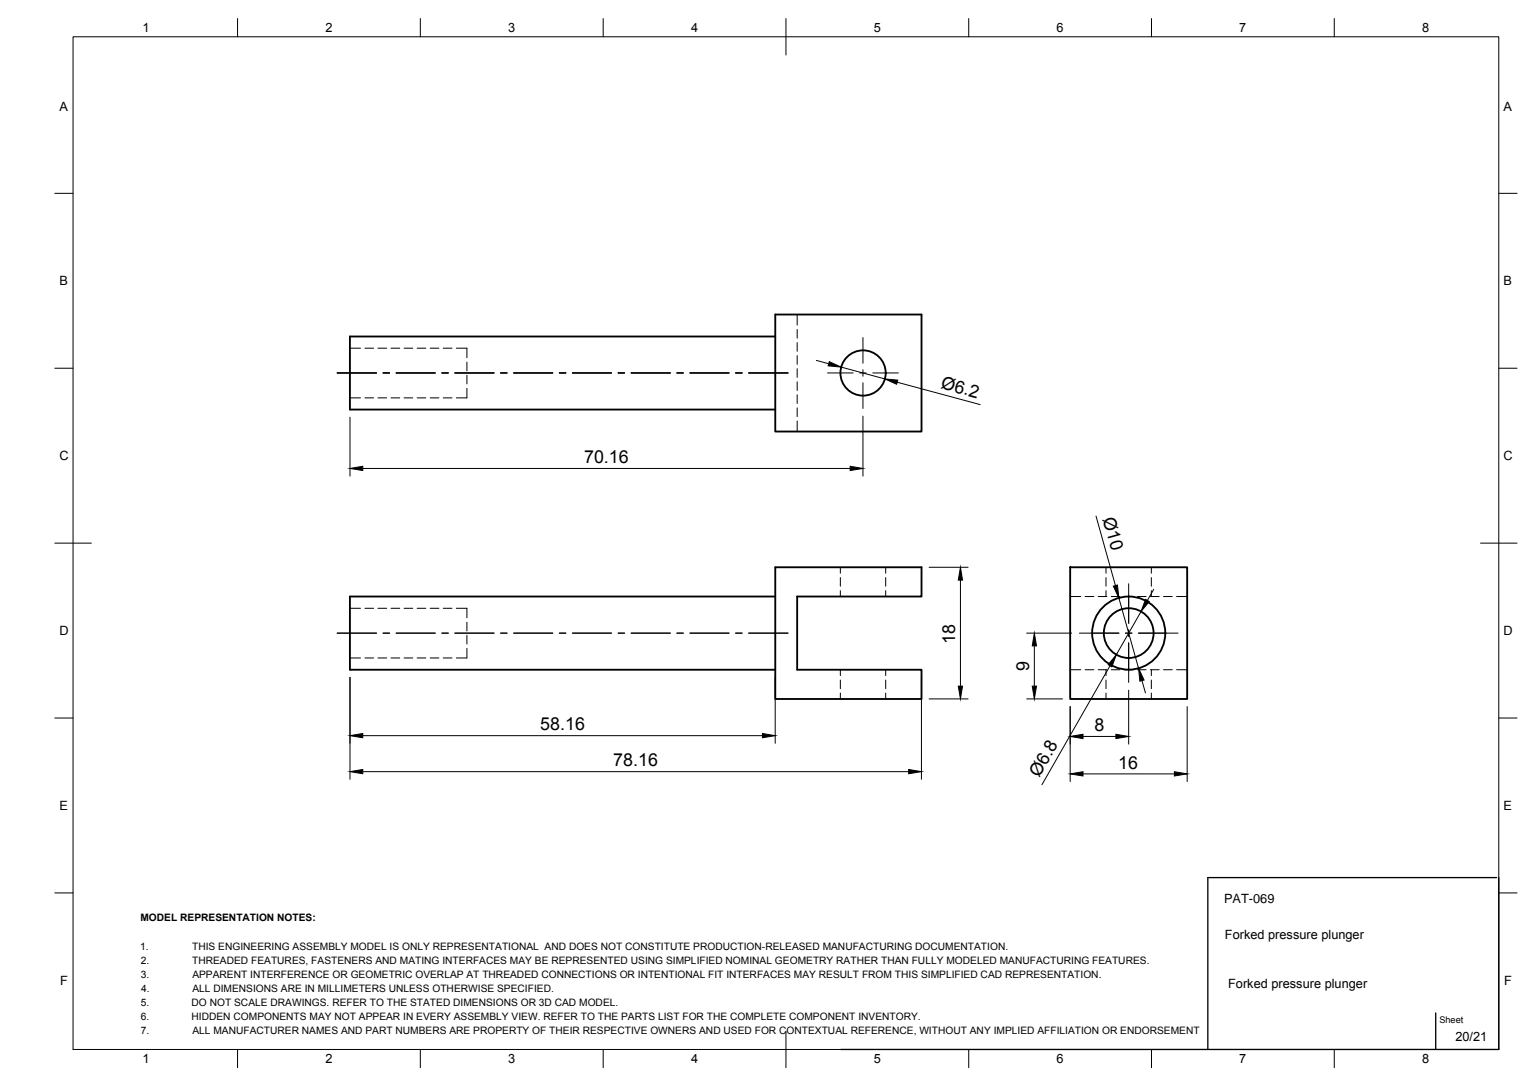
ISO-10303-21;
HEADER;
/* Generated by software containing ST-Developer
 * from STEP Tools, Inc. (www.steptools.com) 
 */

FILE_DESCRIPTION(
/* description */ ('Located fixture plate with toggle clamp'),
/* implementation_level */ '2;1');

FILE_NAME(
/* name */ 'Forked pressure plunger.step',
/* time_stamp */ '2026-10-27T21:36:12-07:00',
/* author */ (''),
/* organization */ (''),
/* preprocessor_version */ 'ST-DEVELOPER v20.2',
/* originating_system */ 'Autodesk Translation Framework v15.17.0.0',
/* authorisation */ '');

FILE_SCHEMA (('AUTOMOTIVE_DESIGN { 1 0 10303 214 3 1 1 }'));
ENDSEC;

DATA;
#10=MECHANICAL_DESIGN_GEOMETRIC_PRESENTATION_REPRESENTATION('',(#337),#9285);
#289=SHAPE_REPRESENTATION_RELATIONSHIP('SRR','None',#9415,#313);
#313=ADVANCED_BREP_SHAPE_REPRESENTATION('',(#358),#9277);
#337=STYLED_ITEM('',(#9598),#358);
#358=MANIFOLD_SOLID_BREP('Body1',#5188);
#470=FACE_BOUND('',#1310,.T.);
#471=FACE_BOUND('',#1313,.T.);
#472=FACE_BOUND('',#1316,.T.);
#473=FACE_BOUND('',#1319,.T.);
#474=FACE_BOUND('',#1322,.T.);
#475=FACE_BOUND('',#1325,.T.);
#632=PLANE('',#5880);
#633=PLANE('',#5887);
#634=PLANE('',#5888);
#635=PLANE('',#5889);
#636=PLANE('',#5890);
#637=PLANE('',#5891);
#638=PLANE('',#5892);
#639=PLANE('',#5894);
#640=PLANE('',#5895);
#641=PLANE('',#5896);
#642=PLANE('',#5897);
#643=PLANE('',#5900);
#905=FACE_OUTER_BOUND('',#1304,.T.);
#906=FACE_OUTER_BOUND('',#1305,.T.);
#907=FACE_OUTER_BOUND('',#1306,.T.);
#908=FACE_OUTER_BOUND('',#1307,.T.);
#909=FACE_OUTER_BOUND('',#1308,.T.);
#910=FACE_OUTER_BOUND('',#1309,.T.);
#911=FACE_OUTER_BOUND('',#1311,.T.);
#912=FACE_OUTER_BOUND('',#1312,.T.);
#913=FACE_OUTER_BOUND('',#1314,.T.);
#914=FACE_OUTER_BOUND('',#1315,.T.);
#915=FACE_OUTER_BOUND('',#1317,.T.);
#916=FACE_OUTER_BOUND('',#1318,.T.);
#917=FACE_OUTER_BOUND('',#1320,.T.);
#918=FACE_OUTER_BOUND('',#1321,.T.);
#919=FACE_OUTER_BOUND('',#1323,.T.);
#920=FACE_OUTER_BOUND('',#1324,.T.);
#1304=EDGE_LOOP('',(#4534,#4535,#4536,#4537));
#1305=EDGE_LOOP('',(#4538));
#1306=EDGE_LOOP('',(#4539,#4540,#4541,#4542));
#1307=EDGE_LOOP('',(#4543,#4544,#4545,#4546));
#1308=EDGE_LOOP('',(#4547,#4548,#4549,#4550));
#1309=EDGE_LOOP('',(#4551,#4552,#4553,#4554));
#1310=EDGE_LOOP('',(#4555));
#1311=EDGE_LOOP('',(#4556,#4557,#4558,#4559,#4560,#4561,#4562,#4563));
#1312=EDGE_LOOP('',(#4564,#4565,#4566,#4567));
#1313=EDGE_LOOP('',(#4568));
#1314=EDGE_LOOP('',(#4569,#4570,#4571,#4572));
#1315=EDGE_LOOP('',(#4573,#4574,#4575,#4576));
#1316=EDGE_LOOP('',(#4577));
#1317=EDGE_LOOP('',(#4578,#4579,#4580,#4581,#4582,#4583,#4584,#4585));
#1318=EDGE_LOOP('',(#4586,#4587,#4588,#4589));
#1319=EDGE_LOOP('',(#4590));
#1320=EDGE_LOOP('',(#4591,#4592,#4593,#4594));
#1321=EDGE_LOOP('',(#4595,#4596,#4597,#4598));
#1322=EDGE_LOOP('',(#4599));
#1323=EDGE_LOOP('',(#4600,#4601,#4602,#4603));
#1324=EDGE_LOOP('',(#4604));
#1325=EDGE_LOOP('',(#4605));
#1544=CIRCLE('',#5878,0.34);
#1545=CIRCLE('',#5879,0.34);
#1546=CIRCLE('',#5882,0.31);
#1547=CIRCLE('',#5883,0.31);
#1548=CIRCLE('',#5885,0.31);
#1549=CIRCLE('',#5886,0.31);
#1550=CIRCLE('',#5893,0.5);
#1551=CIRCLE('',#5899,0.5);
#1923=LINE('',#8748,#2333);
#1924=LINE('',#8755,#2334);
#1925=LINE('',#8761,#2335);
#1926=LINE('',#8766,#2336);
#1927=LINE('',#8768,#2337);
#1928=LINE('',#8770,#2338);
#1929=LINE('',#8771,#2339);
#1930=LINE('',#8775,#2340);
#1931=LINE('',#8777,#2341);
#1932=LINE('',#8779,#2342);
#1933=LINE('',#8780,#2343);
#1934=LINE('',#8783,#2344);
#1935=LINE('',#8784,#2345);
#1936=LINE('',#8786,#2346);
#1937=LINE('',#8788,#2347);
#1938=LINE('',#8790,#2348);
#1939=LINE('',#8791,#2349);
#1940=LINE('',#8795,#2350);
#1941=LINE('',#8796,#2351);
#1942=LINE('',#8797,#2352);
#1943=LINE('',#8800,#2353);
#1944=LINE('',#8801,#2354);
#1945=LINE('',#8803,#2355);
#1946=LINE('',#8807,#2356);
#1947=LINE('',#8809,#2357);
#1948=LINE('',#8810,#2358);
#1949=LINE('',#8813,#2359);
#1950=LINE('',#8818,#2360);
#2333=VECTOR('',#7207,0.34);
#2334=VECTOR('',#7216,0.31);
#2335=VECTOR('',#7223,0.31);
#2336=VECTOR('',#7228,1.);
#2337=VECTOR('',#7229,1.);
#2338=VECTOR('',#7230,1.);
#2339=VECTOR('',#7231,1.);
#2340=VECTOR('',#7234,1.);
#2341=VECTOR('',#7235,1.);
#2342=VECTOR('',#7236,1.);
#2343=VECTOR('',#7237,1.);
#2344=VECTOR('',#7240,1.);
#2345=VECTOR('',#7241,1.);
#2346=VECTOR('',#7242,1.);
#2347=VECTOR('',#7243,1.);
#2348=VECTOR('',#7244,1.);
#2349=VECTOR('',#7245,1.);
#2350=VECTOR('',#7248,1.);
#2351=VECTOR('',#7249,1.);
#2352=VECTOR('',#7250,1.);
#2353=VECTOR('',#7253,1.);
#2354=VECTOR('',#7254,1.);
#2355=VECTOR('',#7257,1.);
#2356=VECTOR('',#7262,1.);
#2357=VECTOR('',#7263,1.);
#2358=VECTOR('',#7264,1.);
#2359=VECTOR('',#7269,1.);
#2360=VECTOR('',#7276,0.5);
#2746=VERTEX_POINT('',#8745);
#2747=VERTEX_POINT('',#8747);
#2748=VERTEX_POINT('',#8752);
#2749=VERTEX_POINT('',#8754);
#2750=VERTEX_POINT('',#8758);
#2751=VERTEX_POINT('',#8760);
#2752=VERTEX_POINT('',#8764);
#2753=VERTEX_POINT('',#8765);
#2754=VERTEX_POINT('',#8767);
#2755=VERTEX_POINT('',#8769);
#2756=VERTEX_POINT('',#8773);
#2757=VERTEX_POINT('',#8774);
#2758=VERTEX_POINT('',#8776);
#2759=VERTEX_POINT('',#8778);
#2760=VERTEX_POINT('',#8782);
#2761=VERTEX_POINT('',#8785);
#2762=VERTEX_POINT('',#8787);
#2763=VERTEX_POINT('',#8789);
#2764=VERTEX_POINT('',#8793);
#2765=VERTEX_POINT('',#8794);
#2766=VERTEX_POINT('',#8799);
#2767=VERTEX_POINT('',#8804);
#2768=VERTEX_POINT('',#8808);
#2769=VERTEX_POINT('',#8816);
#3355=EDGE_CURVE('',#2746,#2746,#1544,.T.);
#3356=EDGE_CURVE('',#2746,#2747,#1923,.T.);
#3357=EDGE_CURVE('',#2747,#2747,#1545,.T.);
#3358=EDGE_CURVE('',#2748,#2748,#1546,.T.);
#3359=EDGE_CURVE('',#2748,#2749,#1924,.T.);
#3360=EDGE_CURVE('',#2749,#2749,#1547,.T.);
#3361=EDGE_CURVE('',#2750,#2750,#1548,.T.);
#3362=EDGE_CURVE('',#2750,#2751,#1925,.T.);
#3363=EDGE_CURVE('',#2751,#2751,#1549,.T.);
#3364=EDGE_CURVE('',#2752,#2753,#1926,.T.);
#3365=EDGE_CURVE('',#2754,#2752,#1927,.T.);
#3366=EDGE_CURVE('',#2755,#2754,#1928,.T.);
#3367=EDGE_CURVE('',#2755,#2753,#1929,.T.);
#3368=EDGE_CURVE('',#2756,#2757,#1930,.T.);
#3369=EDGE_CURVE('',#2757,#2758,#1931,.T.);
#3370=EDGE_CURVE('',#2758,#2759,#1932,.T.);
#3371=EDGE_CURVE('',#2759,#2756,#1933,.T.);
#3372=EDGE_CURVE('',#2760,#2752,#1934,.T.);
#3373=EDGE_CURVE('',#2760,#2757,#1935,.T.);
#3374=EDGE_CURVE('',#2761,#2756,#1936,.T.);
#3375=EDGE_CURVE('',#2762,#2761,#1937,.T.);
#3376=EDGE_CURVE('',#2762,#2763,#1938,.T.);
#3377=EDGE_CURVE('',#2754,#2763,#1939,.T.);
#3378=EDGE_CURVE('',#2764,#2765,#1940,.T.);
#3379=EDGE_CURVE('',#2765,#2762,#1941,.T.);
#3380=EDGE_CURVE('',#2761,#2764,#1942,.T.);
#3381=EDGE_CURVE('',#2766,#2760,#1943,.T.);
#3382=EDGE_CURVE('',#2766,#2758,#1944,.T.);
#3383=EDGE_CURVE('',#2764,#2759,#1945,.T.);
#3384=EDGE_CURVE('',#2767,#2767,#1550,.T.);
#3385=EDGE_CURVE('',#2753,#2766,#1946,.T.);
#3386=EDGE_CURVE('',#2768,#2755,#1947,.T.);
#3387=EDGE_CURVE('',#2765,#2768,#1948,.T.);
#3388=EDGE_CURVE('',#2763,#2768,#1949,.T.);
#3389=EDGE_CURVE('',#2769,#2769,#1551,.T.);
#3390=EDGE_CURVE('',#2769,#2767,#1950,.T.);
#4534=ORIENTED_EDGE('',*,*,#3355,.F.);
#4535=ORIENTED_EDGE('',*,*,#3356,.T.);
#4536=ORIENTED_EDGE('',*,*,#3357,.F.);
#4537=ORIENTED_EDGE('',*,*,#3356,.F.);
#4538=ORIENTED_EDGE('',*,*,#3355,.T.);
#4539=ORIENTED_EDGE('',*,*,#3358,.F.);
#4540=ORIENTED_EDGE('',*,*,#3359,.T.);
#4541=ORIENTED_EDGE('',*,*,#3360,.F.);
#4542=ORIENTED_EDGE('',*,*,#3359,.F.);
#4543=ORIENTED_EDGE('',*,*,#3361,.F.);
#4544=ORIENTED_EDGE('',*,*,#3362,.T.);
#4545=ORIENTED_EDGE('',*,*,#3363,.F.);
#4546=ORIENTED_EDGE('',*,*,#3362,.F.);
#4547=ORIENTED_EDGE('',*,*,#3364,.F.);
#4548=ORIENTED_EDGE('',*,*,#3365,.F.);
#4549=ORIENTED_EDGE('',*,*,#3366,.F.);
#4550=ORIENTED_EDGE('',*,*,#3367,.T.);
#4551=ORIENTED_EDGE('',*,*,#3368,.T.);
#4552=ORIENTED_EDGE('',*,*,#3369,.T.);
#4553=ORIENTED_EDGE('',*,*,#3370,.T.);
#4554=ORIENTED_EDGE('',*,*,#3371,.T.);
#4555=ORIENTED_EDGE('',*,*,#3363,.T.);
#4556=ORIENTED_EDGE('',*,*,#3372,.F.);
#4557=ORIENTED_EDGE('',*,*,#3373,.T.);
#4558=ORIENTED_EDGE('',*,*,#3368,.F.);
#4559=ORIENTED_EDGE('',*,*,#3374,.F.);
#4560=ORIENTED_EDGE('',*,*,#3375,.F.);
#4561=ORIENTED_EDGE('',*,*,#3376,.T.);
#4562=ORIENTED_EDGE('',*,*,#3377,.F.);
#4563=ORIENTED_EDGE('',*,*,#3365,.T.);
#4564=ORIENTED_EDGE('',*,*,#3378,.T.);
#4565=ORIENTED_EDGE('',*,*,#3379,.T.);
#4566=ORIENTED_EDGE('',*,*,#3375,.T.);
#4567=ORIENTED_EDGE('',*,*,#3380,.T.);
#4568=ORIENTED_EDGE('',*,*,#3358,.T.);
#4569=ORIENTED_EDGE('',*,*,#3381,.F.);
#4570=ORIENTED_EDGE('',*,*,#3382,.T.);
#4571=ORIENTED_EDGE('',*,*,#3369,.F.);
#4572=ORIENTED_EDGE('',*,*,#3373,.F.);
#4573=ORIENTED_EDGE('',*,*,#3374,.T.);
#4574=ORIENTED_EDGE('',*,*,#3371,.F.);
#4575=ORIENTED_EDGE('',*,*,#3383,.F.);
#4576=ORIENTED_EDGE('',*,*,#3380,.F.);
#4577=ORIENTED_EDGE('',*,*,#3384,.F.);
#4578=ORIENTED_EDGE('',*,*,#3370,.F.);
#4579=ORIENTED_EDGE('',*,*,#3382,.F.);
#4580=ORIENTED_EDGE('',*,*,#3385,.F.);
#4581=ORIENTED_EDGE('',*,*,#3367,.F.);
#4582=ORIENTED_EDGE('',*,*,#3386,.F.);
#4583=ORIENTED_EDGE('',*,*,#3387,.F.);
#4584=ORIENTED_EDGE('',*,*,#3378,.F.);
#4585=ORIENTED_EDGE('',*,*,#3383,.T.);
#4586=ORIENTED_EDGE('',*,*,#3364,.T.);
#4587=ORIENTED_EDGE('',*,*,#3385,.T.);
#4588=ORIENTED_EDGE('',*,*,#3381,.T.);
#4589=ORIENTED_EDGE('',*,*,#3372,.T.);
#4590=ORIENTED_EDGE('',*,*,#3361,.T.);
#4591=ORIENTED_EDGE('',*,*,#3379,.F.);
#4592=ORIENTED_EDGE('',*,*,#3387,.T.);
#4593=ORIENTED_EDGE('',*,*,#3388,.F.);
#4594=ORIENTED_EDGE('',*,*,#3376,.F.);
#4595=ORIENTED_EDGE('',*,*,#3366,.T.);
#4596=ORIENTED_EDGE('',*,*,#3377,.T.);
#4597=ORIENTED_EDGE('',*,*,#3388,.T.);
#4598=ORIENTED_EDGE('',*,*,#3386,.T.);
#4599=ORIENTED_EDGE('',*,*,#3360,.T.);
#4600=ORIENTED_EDGE('',*,*,#3389,.F.);
#4601=ORIENTED_EDGE('',*,*,#3390,.T.);
#4602=ORIENTED_EDGE('',*,*,#3384,.T.);
#4603=ORIENTED_EDGE('',*,*,#3390,.F.);
#4604=ORIENTED_EDGE('',*,*,#3389,.T.);
#4605=ORIENTED_EDGE('',*,*,#3357,.T.);
#4859=CYLINDRICAL_SURFACE('',#5877,0.34);
#4860=CYLINDRICAL_SURFACE('',#5881,0.31);
#4861=CYLINDRICAL_SURFACE('',#5884,0.31);
#4862=CYLINDRICAL_SURFACE('',#5898,0.5);
#5106=ADVANCED_FACE('',(#905),#4859,.F.);
#5107=ADVANCED_FACE('',(#906),#632,.T.);
#5108=ADVANCED_FACE('',(#907),#4860,.F.);
#5109=ADVANCED_FACE('',(#908),#4861,.F.);
#5110=ADVANCED_FACE('',(#909),#633,.T.);
#5111=ADVANCED_FACE('',(#910,#470),#634,.T.);
#5112=ADVANCED_FACE('',(#911),#635,.T.);
#5113=ADVANCED_FACE('',(#912,#471),#636,.F.);
#5114=ADVANCED_FACE('',(#913),#637,.T.);
#5115=ADVANCED_FACE('',(#914,#472),#638,.T.);
#5116=ADVANCED_FACE('',(#915),#639,.T.);
#5117=ADVANCED_FACE('',(#916,#473),#640,.F.);
#5118=ADVANCED_FACE('',(#917),#641,.T.);
#5119=ADVANCED_FACE('',(#918,#474),#642,.T.);
#5120=ADVANCED_FACE('',(#919),#4862,.T.);
#5121=ADVANCED_FACE('',(#920,#475),#643,.T.);
#5188=CLOSED_SHELL('',(#5106,#5107,#5108,#5109,#5110,#5111,#5112,#5113,
#5114,#5115,#5116,#5117,#5118,#5119,#5120,#5121));
#5876=AXIS2_PLACEMENT_3D('',#8743,#7201,#7202);
#5877=AXIS2_PLACEMENT_3D('',#8744,#7203,#7204);
#5878=AXIS2_PLACEMENT_3D('',#8746,#7205,#7206);
#5879=AXIS2_PLACEMENT_3D('',#8749,#7208,#7209);
#5880=AXIS2_PLACEMENT_3D('',#8750,#7210,#7211);
#5881=AXIS2_PLACEMENT_3D('',#8751,#7212,#7213);
#5882=AXIS2_PLACEMENT_3D('',#8753,#7214,#7215);
#5883=AXIS2_PLACEMENT_3D('',#8756,#7217,#7218);
#5884=AXIS2_PLACEMENT_3D('',#8757,#7219,#7220);
#5885=AXIS2_PLACEMENT_3D('',#8759,#7221,#7222);
#5886=AXIS2_PLACEMENT_3D('',#8762,#7224,#7225);
#5887=AXIS2_PLACEMENT_3D('',#8763,#7226,#7227);
#5888=AXIS2_PLACEMENT_3D('',#8772,#7232,#7233);
#5889=AXIS2_PLACEMENT_3D('',#8781,#7238,#7239);
#5890=AXIS2_PLACEMENT_3D('',#8792,#7246,#7247);
#5891=AXIS2_PLACEMENT_3D('',#8798,#7251,#7252);
#5892=AXIS2_PLACEMENT_3D('',#8802,#7255,#7256);
#5893=AXIS2_PLACEMENT_3D('',#8805,#7258,#7259);
#5894=AXIS2_PLACEMENT_3D('',#8806,#7260,#7261);
#5895=AXIS2_PLACEMENT_3D('',#8811,#7265,#7266);
#5896=AXIS2_PLACEMENT_3D('',#8812,#7267,#7268);
#5897=AXIS2_PLACEMENT_3D('',#8814,#7270,#7271);
#5898=AXIS2_PLACEMENT_3D('',#8815,#7272,#7273);
#5899=AXIS2_PLACEMENT_3D('',#8817,#7274,#7275);
#5900=AXIS2_PLACEMENT_3D('',#8819,#7277,#7278);
#7201=DIRECTION('axis',(0.,0.,1.));
#7202=DIRECTION('refdir',(1.,0.,0.));
#7203=DIRECTION('center_axis',(1.,0.,0.));
#7204=DIRECTION('ref_axis',(0.,0.,-1.));
#7205=DIRECTION('center_axis',(1.,0.,0.));
#7206=DIRECTION('ref_axis',(0.,0.,-1.));
#7207=DIRECTION('',(1.,0.,0.));
#7208=DIRECTION('center_axis',(-1.,0.,0.));
#7209=DIRECTION('ref_axis',(0.,0.,-1.));
#7210=DIRECTION('center_axis',(1.,0.,0.));
#7211=DIRECTION('ref_axis',(0.,0.,-1.));
#7212=DIRECTION('center_axis',(0.,1.,0.));
#7213=DIRECTION('ref_axis',(1.,0.,0.));
#7214=DIRECTION('center_axis',(0.,1.,0.));
#7215=DIRECTION('ref_axis',(1.,0.,0.));
#7216=DIRECTION('',(0.,1.,0.));
#7217=DIRECTION('center_axis',(0.,-1.,0.));
#7218=DIRECTION('ref_axis',(1.,0.,0.));
#7219=DIRECTION('center_axis',(0.,1.,0.));
#7220=DIRECTION('ref_axis',(1.,0.,0.));
#7221=DIRECTION('center_axis',(0.,1.,0.));
#7222=DIRECTION('ref_axis',(1.,0.,0.));
#7223=DIRECTION('',(0.,1.,0.));
#7224=DIRECTION('center_axis',(0.,-1.,0.));
#7225=DIRECTION('ref_axis',(1.,0.,0.));
#7226=DIRECTION('center_axis',(-1.,0.,0.));
#7227=DIRECTION('ref_axis',(0.,0.,1.));
#7228=DIRECTION('',(0.,0.,1.));
#7229=DIRECTION('',(0.,1.,0.));
#7230=DIRECTION('',(0.,0.,-1.));
#7231=DIRECTION('',(0.,1.,0.));
#7232=DIRECTION('center_axis',(0.,1.,0.));
#7233=DIRECTION('ref_axis',(0.,0.,1.));
#7234=DIRECTION('',(-1.,0.,0.));
#7235=DIRECTION('',(0.,0.,1.));
#7236=DIRECTION('',(1.,0.,0.));
#7237=DIRECTION('',(0.,0.,-1.));
#7238=DIRECTION('center_axis',(0.,0.,-1.));
#7239=DIRECTION('ref_axis',(-1.,0.,0.));
#7240=DIRECTION('',(1.,0.,0.));
#7241=DIRECTION('',(0.,1.,0.));
#7242=DIRECTION('',(0.,1.,0.));
#7243=DIRECTION('',(1.,0.,0.));
#7244=DIRECTION('',(0.,1.,0.));
#7245=DIRECTION('',(-1.,0.,0.));
#7246=DIRECTION('center_axis',(0.,1.,0.));
#7247=DIRECTION('ref_axis',(1.,0.,0.));
#7248=DIRECTION('',(-1.,0.,0.));
#7249=DIRECTION('',(0.,0.,-1.));
#7250=DIRECTION('',(0.,0.,1.));
#7251=DIRECTION('center_axis',(-1.,0.,0.));
#7252=DIRECTION('ref_axis',(0.,0.,1.));
#7253=DIRECTION('',(0.,0.,-1.));
#7254=DIRECTION('',(0.,1.,0.));
#7255=DIRECTION('center_axis',(1.,0.,0.));
#7256=DIRECTION('ref_axis',(0.,0.,-1.));
#7257=DIRECTION('',(0.,1.,0.));
#7258=DIRECTION('center_axis',(1.,0.,0.));
#7259=DIRECTION('ref_axis',(0.,0.,-1.));
#7260=DIRECTION('center_axis',(0.,0.,1.));
#7261=DIRECTION('ref_axis',(1.,0.,0.));
#7262=DIRECTION('',(-1.,0.,0.));
#7263=DIRECTION('',(1.,0.,0.));
#7264=DIRECTION('',(0.,1.,0.));
#7265=DIRECTION('center_axis',(0.,1.,0.));
#7266=DIRECTION('ref_axis',(1.,0.,0.));
#7267=DIRECTION('center_axis',(-1.,0.,0.));
#7268=DIRECTION('ref_axis',(0.,0.,1.));
#7269=DIRECTION('',(0.,0.,1.));
#7270=DIRECTION('center_axis',(0.,1.,0.));
#7271=DIRECTION('ref_axis',(0.,0.,1.));
#7272=DIRECTION('center_axis',(1.,0.,0.));
#7273=DIRECTION('ref_axis',(0.,0.,-1.));
#7274=DIRECTION('center_axis',(1.,0.,0.));
#7275=DIRECTION('ref_axis',(0.,0.,-1.));
#7276=DIRECTION('',(-1.,0.,0.));
#7277=DIRECTION('center_axis',(1.,0.,0.));
#7278=DIRECTION('ref_axis',(0.,0.,-1.));
#8743=CARTESIAN_POINT('',(0.,0.,0.));
#8744=CARTESIAN_POINT('Origin',(11.4,0.,2.5));
#8745=CARTESIAN_POINT('',(11.4,-4.163799117101E-17,2.84));
#8746=CARTESIAN_POINT('Origin',(11.4,0.,2.5));
#8747=CARTESIAN_POINT('',(13.,4.163799117101E-17,2.84));
#8748=CARTESIAN_POINT('',(11.4,-4.163799117101E-17,2.84));
#8749=CARTESIAN_POINT('Origin',(13.,0.,2.5));
#8750=CARTESIAN_POINT('Origin',(11.4,0.,2.5));
#8751=CARTESIAN_POINT('Origin',(5.98369790806552,-1.,2.5));
#8752=CARTESIAN_POINT('',(5.67369790806552,-0.9,2.5));
#8753=CARTESIAN_POINT('Origin',(5.98369790806552,-0.9,2.5));
#8754=CARTESIAN_POINT('',(5.67369790806552,-0.5,2.5));
#8755=CARTESIAN_POINT('',(5.67369790806552,-1.,2.5));
#8756=CARTESIAN_POINT('Origin',(5.98369790806552,-0.5,2.5));
#8757=CARTESIAN_POINT('Origin',(5.98369790806552,-1.,2.5));
#8758=CARTESIAN_POINT('',(5.67369790806552,0.5,2.5));
#8759=CARTESIAN_POINT('Origin',(5.98369790806552,0.5,2.5));
#8760=CARTESIAN_POINT('',(5.67369790806552,0.9,2.5));
#8761=CARTESIAN_POINT('',(5.67369790806552,-1.,2.5));
#8762=CARTESIAN_POINT('Origin',(5.98369790806552,0.9,2.5));
#8763=CARTESIAN_POINT('Origin',(6.88369790806552,-0.9,1.7));
#8764=CARTESIAN_POINT('',(6.88369790806552,0.5,1.7));
#8765=CARTESIAN_POINT('',(6.88369790806552,0.5,3.3));
#8766=CARTESIAN_POINT('',(6.88369790806552,0.5,2.1));
#8767=CARTESIAN_POINT('',(6.88369790806552,-0.5,1.7));
#8768=CARTESIAN_POINT('',(6.88369790806552,-0.9,1.7));
#8769=CARTESIAN_POINT('',(6.88369790806552,-0.5,3.3));
#8770=CARTESIAN_POINT('',(6.88369790806552,-0.5,2.1));
#8771=CARTESIAN_POINT('',(6.88369790806552,-0.9,3.3));
#8772=CARTESIAN_POINT('Origin',(6.18369790806552,0.9,2.5));
#8773=CARTESIAN_POINT('',(7.18369790806552,0.9,1.7));
#8774=CARTESIAN_POINT('',(5.18369790806552,0.9,1.7));
#8775=CARTESIAN_POINT('',(5.18369790806552,0.9,1.7));
#8776=CARTESIAN_POINT('',(5.18369790806552,0.9,3.3));
#8777=CARTESIAN_POINT('',(5.18369790806552,0.9,3.3));
#8778=CARTESIAN_POINT('',(7.18369790806552,0.9,3.3));
#8779=CARTESIAN_POINT('',(7.18369790806552,0.9,3.3));
#8780=CARTESIAN_POINT('',(7.18369790806552,0.9,1.7));
#8781=CARTESIAN_POINT('Origin',(7.18369790806552,0.5,1.7));
#8782=CARTESIAN_POINT('',(5.18369790806552,0.5,1.7));
#8783=CARTESIAN_POINT('',(5.18369790806552,0.5,1.7));
#8784=CARTESIAN_POINT('',(5.18369790806552,0.5,1.7));
#8785=CARTESIAN_POINT('',(7.18369790806552,-0.9,1.7));
#8786=CARTESIAN_POINT('',(7.18369790806552,0.5,1.7));
#8787=CARTESIAN_POINT('',(5.18369790806552,-0.9,1.7));
#8788=CARTESIAN_POINT('',(5.18369790806552,-0.9,1.7));
#8789=CARTESIAN_POINT('',(5.18369790806552,-0.5,1.7));
#8790=CARTESIAN_POINT('',(5.18369790806552,-0.9,1.7));
#8791=CARTESIAN_POINT('',(5.18369790806552,-0.5,1.7));
#8792=CARTESIAN_POINT('Origin',(6.18369790806552,-0.9,2.5));
#8793=CARTESIAN_POINT('',(7.18369790806552,-0.9,3.3));
#8794=CARTESIAN_POINT('',(5.18369790806552,-0.9,3.3));
#8795=CARTESIAN_POINT('',(7.18369790806552,-0.9,3.3));
#8796=CARTESIAN_POINT('',(5.18369790806552,-0.9,3.3));
#8797=CARTESIAN_POINT('',(7.18369790806552,-0.9,1.7));
#8798=CARTESIAN_POINT('Origin',(5.18369790806552,0.5,1.7));
#8799=CARTESIAN_POINT('',(5.18369790806552,0.5,3.3));
#8800=CARTESIAN_POINT('',(5.18369790806552,0.5,3.3));
#8801=CARTESIAN_POINT('',(5.18369790806552,0.5,3.3));
#8802=CARTESIAN_POINT('Origin',(7.18369790806552,0.5,3.3));
#8803=CARTESIAN_POINT('',(7.18369790806552,0.5,3.3));
#8804=CARTESIAN_POINT('',(7.18369790806552,-6.12323399573677E-17,3.));
#8805=CARTESIAN_POINT('Origin',(7.18369790806552,0.,2.5));
#8806=CARTESIAN_POINT('Origin',(5.18369790806552,0.5,3.3));
#8807=CARTESIAN_POINT('',(7.18369790806552,0.5,3.3));
#8808=CARTESIAN_POINT('',(5.18369790806552,-0.5,3.3));
#8809=CARTESIAN_POINT('',(7.18369790806552,-0.5,3.3));
#8810=CARTESIAN_POINT('',(5.18369790806552,-0.9,3.3));
#8811=CARTESIAN_POINT('Origin',(6.18369790806552,0.5,2.5));
#8812=CARTESIAN_POINT('Origin',(5.18369790806552,-0.9,1.7));
#8813=CARTESIAN_POINT('',(5.18369790806552,-0.5,3.3));
#8814=CARTESIAN_POINT('Origin',(6.18369790806552,-0.5,2.5));
#8815=CARTESIAN_POINT('Origin',(6.98369791,0.,2.5));
#8816=CARTESIAN_POINT('',(13.,-6.12323399573677E-17,3.));
#8817=CARTESIAN_POINT('Origin',(13.,0.,2.5));
#8818=CARTESIAN_POINT('',(6.98369791,-6.12323399573677E-17,3.));
#8819=CARTESIAN_POINT('Origin',(13.,0.,2.5));
#9247=UNCERTAINTY_MEASURE_WITH_UNIT(LENGTH_MEASURE(0.001),#9286,
'DISTANCE_ACCURACY_VALUE',
'Maximum model space distance between geometric entities at asserted c
onnectivities');
#9255=UNCERTAINTY_MEASURE_WITH_UNIT(LENGTH_MEASURE(0.001),#9286,
'DISTANCE_ACCURACY_VALUE',
'Maximum model space distance between geometric entities at asserted c
onnectivities');
#9277=(
GEOMETRIC_REPRESENTATION_CONTEXT(3)
GLOBAL_UNCERTAINTY_ASSIGNED_CONTEXT((#9247))
GLOBAL_UNIT_ASSIGNED_CONTEXT((#9286,#9288,#9289))
REPRESENTATION_CONTEXT('','3D')
);
#9285=(
GEOMETRIC_REPRESENTATION_CONTEXT(3)
GLOBAL_UNCERTAINTY_ASSIGNED_CONTEXT((#9255))
GLOBAL_UNIT_ASSIGNED_CONTEXT((#9286,#9288,#9289))
REPRESENTATION_CONTEXT('','3D')
);
#9286=(
LENGTH_UNIT()
NAMED_UNIT(*)
SI_UNIT(.CENTI.,.METRE.)
);
#9288=(
NAMED_UNIT(*)
PLANE_ANGLE_UNIT()
SI_UNIT($,.RADIAN.)
);
#9289=(
NAMED_UNIT(*)
SI_UNIT($,.STERADIAN.)
SOLID_ANGLE_UNIT()
);
#9311=SHAPE_DEFINITION_REPRESENTATION(#9341,#9415);
#9341=PRODUCT_DEFINITION_SHAPE('',$,#9445);
#9415=SHAPE_REPRESENTATION('',(#5876),#9277);
#9423=PRODUCT_DEFINITION_CONTEXT('part definition',#9512,'design');
#9445=PRODUCT_DEFINITION('Forked pressure plunger',
'Forked pressure plunger',#9474,#9423);
#9474=PRODUCT_DEFINITION_FORMATION('',$,#9535);
#9512=APPLICATION_CONTEXT(
'Core Data for Automotive Mechanical Design Process');
#9513=PRODUCT_CONTEXT('part definition',#9512,'mechanical');
#9535=PRODUCT('Forked pressure plunger','Forked pressure plunger',
'Forked pressure plunger',(#9513));
#9592=COLOUR_RGB('Light Blue',0.38,0.62,0.78);
#9593=FILL_AREA_STYLE_COLOUR('',#9592);
#9594=FILL_AREA_STYLE('',(#9593));
#9595=SURFACE_STYLE_FILL_AREA(#9594);
#9596=SURFACE_SIDE_STYLE('',(#9595));
#9597=SURFACE_STYLE_USAGE(.BOTH.,#9596);
#9598=PRESENTATION_STYLE_ASSIGNMENT((#9597));
ENDSEC;
END-ISO-10303-21;
